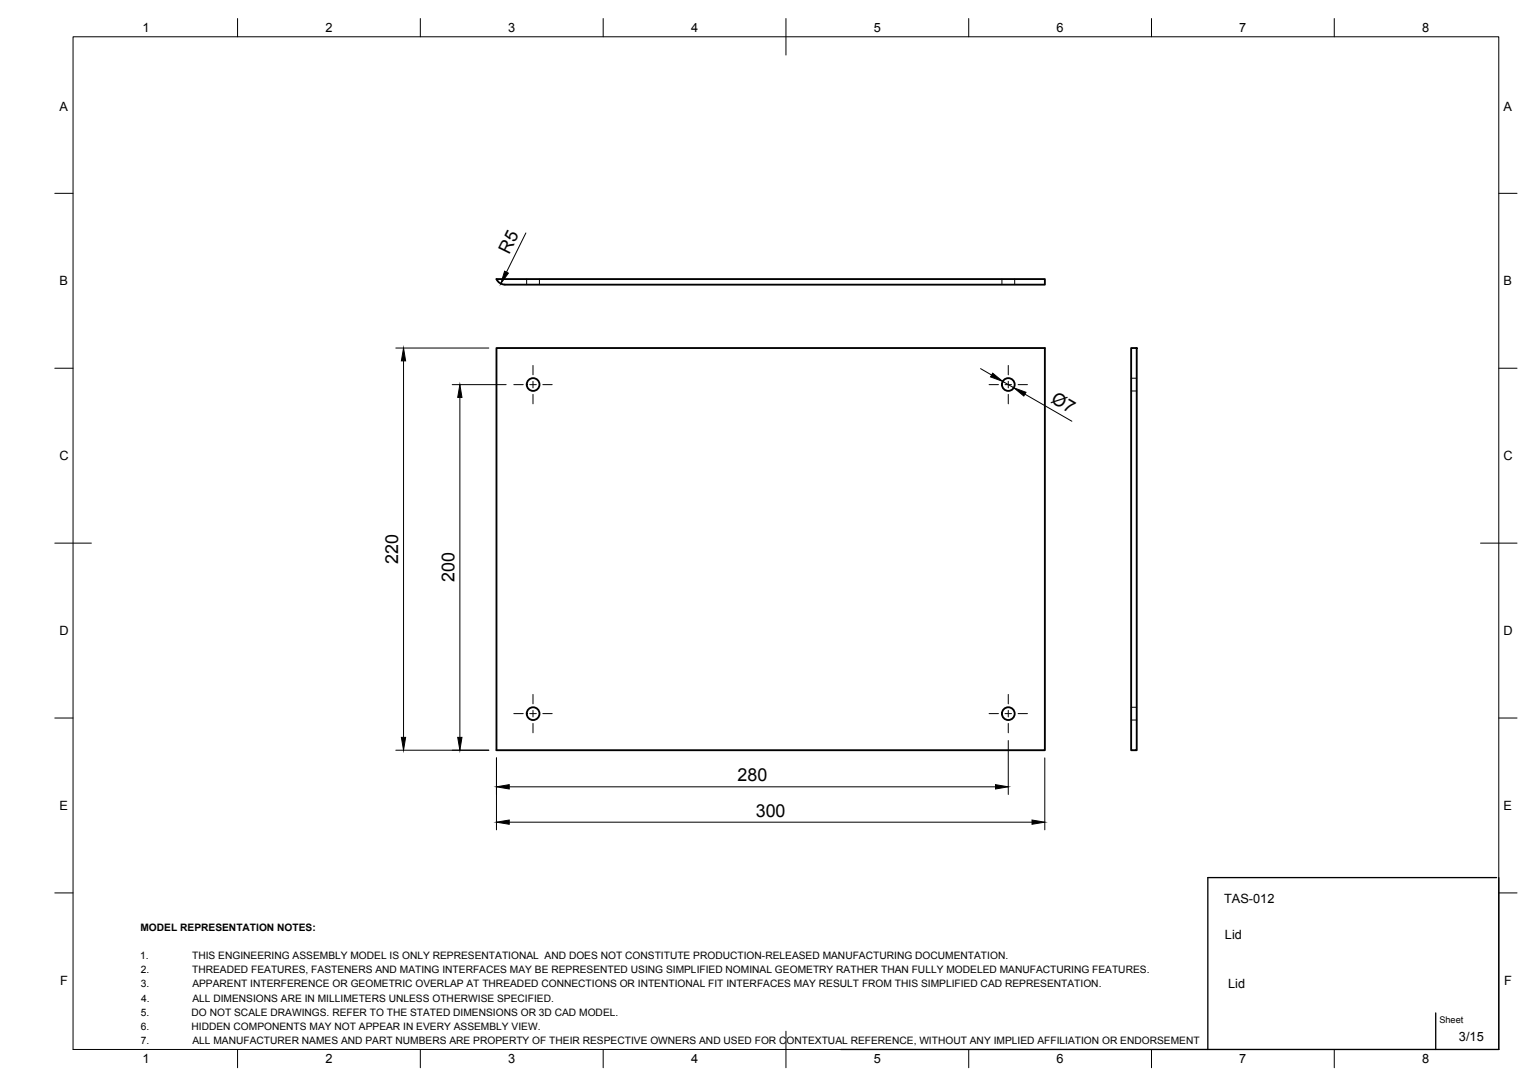
ISO-10303-21;
HEADER;
/* Generated by software containing ST-Developer
 * from STEP Tools, Inc. (www.steptools.com) 
 */

FILE_DESCRIPTION(
/* description */ (
'Independent welded steel electronics enclosure with removable sealed 
lid, internal mounting tray and two threaded cable entries. 300 x 220 
mm body. No ingress or electrical safety rating assigned.'),
/* implementation_level */ '2;1');

FILE_NAME(
/* name */ 'Lid.step',
/* time_stamp */ '2026-11-14T09:13:27-08:00',
/* author */ (''),
/* organization */ (''),
/* preprocessor_version */ 'ST-DEVELOPER v20.2',
/* originating_system */ 'Autodesk Translation Framework v15.17.0.0',
/* authorisation */ '');

FILE_SCHEMA (('AUTOMOTIVE_DESIGN { 1 0 10303 214 3 1 1 }'));
ENDSEC;

DATA;
#10=MECHANICAL_DESIGN_GEOMETRIC_PRESENTATION_REPRESENTATION('',(#973),#94412);
#943=SHAPE_REPRESENTATION_RELATIONSHIP('SRR','None',#94495,#958);
#958=ADVANCED_BREP_SHAPE_REPRESENTATION('',(#988),#94404);
#973=STYLED_ITEM('',(#94579),#988);
#988=MANIFOLD_SOLID_BREP('Body1',#8258);
#1017=FACE_BOUND('',#1741,.T.);
#1018=FACE_BOUND('',#1742,.T.);
#1019=FACE_BOUND('',#1743,.T.);
#1020=FACE_BOUND('',#1744,.T.);
#1021=FACE_BOUND('',#1753,.T.);
#1022=FACE_BOUND('',#1754,.T.);
#1023=FACE_BOUND('',#1755,.T.);
#1024=FACE_BOUND('',#1756,.T.);
#1110=PLANE('',#8714);
#1111=PLANE('',#8719);
#1112=PLANE('',#8728);
#1113=PLANE('',#8729);
#1114=PLANE('',#8730);
#1362=FACE_OUTER_BOUND('',#1739,.T.);
#1363=FACE_OUTER_BOUND('',#1740,.T.);
#1364=FACE_OUTER_BOUND('',#1745,.T.);
#1365=FACE_OUTER_BOUND('',#1746,.T.);
#1366=FACE_OUTER_BOUND('',#1747,.T.);
#1367=FACE_OUTER_BOUND('',#1748,.T.);
#1368=FACE_OUTER_BOUND('',#1749,.T.);
#1369=FACE_OUTER_BOUND('',#1750,.T.);
#1370=FACE_OUTER_BOUND('',#1751,.T.);
#1371=FACE_OUTER_BOUND('',#1752,.T.);
#1739=EDGE_LOOP('',(#6644,#6645,#6646,#6647));
#1740=EDGE_LOOP('',(#6648,#6649,#6650,#6651));
#1741=EDGE_LOOP('',(#6652));
#1742=EDGE_LOOP('',(#6653));
#1743=EDGE_LOOP('',(#6654));
#1744=EDGE_LOOP('',(#6655));
#1745=EDGE_LOOP('',(#6656,#6657,#6658,#6659));
#1746=EDGE_LOOP('',(#6660,#6661,#6662,#6663));
#1747=EDGE_LOOP('',(#6664,#6665,#6666,#6667));
#1748=EDGE_LOOP('',(#6668,#6669,#6670,#6671));
#1749=EDGE_LOOP('',(#6672,#6673,#6674,#6675));
#1750=EDGE_LOOP('',(#6676,#6677,#6678,#6679));
#1751=EDGE_LOOP('',(#6680,#6681,#6682,#6683));
#1752=EDGE_LOOP('',(#6684,#6685,#6686,#6687));
#1753=EDGE_LOOP('',(#6688));
#1754=EDGE_LOOP('',(#6689));
#1755=EDGE_LOOP('',(#6690));
#1756=EDGE_LOOP('',(#6691));
#2161=LINE('',#59703,#2559);
#2162=LINE('',#59706,#2560);
#2163=LINE('',#59709,#2561);
#2164=LINE('',#59711,#2562);
#2165=LINE('',#59712,#2563);
#2166=LINE('',#59723,#2564);
#2167=LINE('',#59724,#2565);
#2168=LINE('',#59727,#2566);
#2169=LINE('',#59731,#2567);
#2170=LINE('',#59735,#2568);
#2171=LINE('',#59739,#2569);
#2172=LINE('',#59743,#2570);
#2173=LINE('',#59744,#2571);
#2174=LINE('',#59746,#2572);
#2559=VECTOR('',#9733,5.);
#2560=VECTOR('',#9736,10.);
#2561=VECTOR('',#9739,10.);
#2562=VECTOR('',#9740,10.);
#2563=VECTOR('',#9741,10.);
#2564=VECTOR('',#9752,10.);
#2565=VECTOR('',#9753,10.);
#2566=VECTOR('',#9756,3.5);
#2567=VECTOR('',#9761,3.5);
#2568=VECTOR('',#9766,3.5);
#2569=VECTOR('',#9771,3.5);
#2570=VECTOR('',#9776,10.);
#2571=VECTOR('',#9777,10.);
#2572=VECTOR('',#9780,10.);
#2784=CIRCLE('',#8712,5.00000000000001);
#2785=CIRCLE('',#8713,5.00000000000001);
#2786=CIRCLE('',#8715,3.5);
#2787=CIRCLE('',#8716,3.5);
#2788=CIRCLE('',#8717,3.5);
#2789=CIRCLE('',#8718,3.5);
#2790=CIRCLE('',#8721,3.5);
#2791=CIRCLE('',#8723,3.5);
#2792=CIRCLE('',#8725,3.5);
#2793=CIRCLE('',#8727,3.5);
#3436=VERTEX_POINT('',#59699);
#3437=VERTEX_POINT('',#59700);
#3438=VERTEX_POINT('',#59702);
#3439=VERTEX_POINT('',#59704);
#3440=VERTEX_POINT('',#59708);
#3441=VERTEX_POINT('',#59710);
#3442=VERTEX_POINT('',#59713);
#3443=VERTEX_POINT('',#59715);
#3444=VERTEX_POINT('',#59717);
#3445=VERTEX_POINT('',#59719);
#3446=VERTEX_POINT('',#59722);
#3447=VERTEX_POINT('',#59726);
#3448=VERTEX_POINT('',#59730);
#3449=VERTEX_POINT('',#59734);
#3450=VERTEX_POINT('',#59738);
#3451=VERTEX_POINT('',#59742);
#4587=EDGE_CURVE('',#3436,#3437,#2784,.T.);
#4588=EDGE_CURVE('',#3437,#3438,#2161,.T.);
#4589=EDGE_CURVE('',#3438,#3439,#2785,.T.);
#4590=EDGE_CURVE('',#3439,#3436,#2162,.T.);
#4591=EDGE_CURVE('',#3437,#3440,#2163,.T.);
#4592=EDGE_CURVE('',#3440,#3441,#2164,.T.);
#4593=EDGE_CURVE('',#3441,#3438,#2165,.T.);
#4594=EDGE_CURVE('',#3442,#3442,#2786,.T.);
#4595=EDGE_CURVE('',#3443,#3443,#2787,.T.);
#4596=EDGE_CURVE('',#3444,#3444,#2788,.T.);
#4597=EDGE_CURVE('',#3445,#3445,#2789,.T.);
#4598=EDGE_CURVE('',#3436,#3446,#2166,.T.);
#4599=EDGE_CURVE('',#3446,#3440,#2167,.T.);
#4600=EDGE_CURVE('',#3445,#3447,#2168,.T.);
#4601=EDGE_CURVE('',#3447,#3447,#2790,.T.);
#4602=EDGE_CURVE('',#3444,#3448,#2169,.T.);
#4603=EDGE_CURVE('',#3448,#3448,#2791,.T.);
#4604=EDGE_CURVE('',#3443,#3449,#2170,.T.);
#4605=EDGE_CURVE('',#3449,#3449,#2792,.T.);
#4606=EDGE_CURVE('',#3442,#3450,#2171,.T.);
#4607=EDGE_CURVE('',#3450,#3450,#2793,.T.);
#4608=EDGE_CURVE('',#3451,#3441,#2172,.T.);
#4609=EDGE_CURVE('',#3451,#3439,#2173,.T.);
#4610=EDGE_CURVE('',#3446,#3451,#2174,.T.);
#6644=ORIENTED_EDGE('',*,*,#4587,.T.);
#6645=ORIENTED_EDGE('',*,*,#4588,.T.);
#6646=ORIENTED_EDGE('',*,*,#4589,.T.);
#6647=ORIENTED_EDGE('',*,*,#4590,.T.);
#6648=ORIENTED_EDGE('',*,*,#4588,.F.);
#6649=ORIENTED_EDGE('',*,*,#4591,.T.);
#6650=ORIENTED_EDGE('',*,*,#4592,.T.);
#6651=ORIENTED_EDGE('',*,*,#4593,.T.);
#6652=ORIENTED_EDGE('',*,*,#4594,.T.);
#6653=ORIENTED_EDGE('',*,*,#4595,.T.);
#6654=ORIENTED_EDGE('',*,*,#4596,.T.);
#6655=ORIENTED_EDGE('',*,*,#4597,.T.);
#6656=ORIENTED_EDGE('',*,*,#4587,.F.);
#6657=ORIENTED_EDGE('',*,*,#4598,.T.);
#6658=ORIENTED_EDGE('',*,*,#4599,.T.);
#6659=ORIENTED_EDGE('',*,*,#4591,.F.);
#6660=ORIENTED_EDGE('',*,*,#4597,.F.);
#6661=ORIENTED_EDGE('',*,*,#4600,.T.);
#6662=ORIENTED_EDGE('',*,*,#4601,.F.);
#6663=ORIENTED_EDGE('',*,*,#4600,.F.);
#6664=ORIENTED_EDGE('',*,*,#4596,.F.);
#6665=ORIENTED_EDGE('',*,*,#4602,.T.);
#6666=ORIENTED_EDGE('',*,*,#4603,.F.);
#6667=ORIENTED_EDGE('',*,*,#4602,.F.);
#6668=ORIENTED_EDGE('',*,*,#4595,.F.);
#6669=ORIENTED_EDGE('',*,*,#4604,.T.);
#6670=ORIENTED_EDGE('',*,*,#4605,.F.);
#6671=ORIENTED_EDGE('',*,*,#4604,.F.);
#6672=ORIENTED_EDGE('',*,*,#4594,.F.);
#6673=ORIENTED_EDGE('',*,*,#4606,.T.);
#6674=ORIENTED_EDGE('',*,*,#4607,.F.);
#6675=ORIENTED_EDGE('',*,*,#4606,.F.);
#6676=ORIENTED_EDGE('',*,*,#4589,.F.);
#6677=ORIENTED_EDGE('',*,*,#4593,.F.);
#6678=ORIENTED_EDGE('',*,*,#4608,.F.);
#6679=ORIENTED_EDGE('',*,*,#4609,.T.);
#6680=ORIENTED_EDGE('',*,*,#4610,.T.);
#6681=ORIENTED_EDGE('',*,*,#4608,.T.);
#6682=ORIENTED_EDGE('',*,*,#4592,.F.);
#6683=ORIENTED_EDGE('',*,*,#4599,.F.);
#6684=ORIENTED_EDGE('',*,*,#4610,.F.);
#6685=ORIENTED_EDGE('',*,*,#4598,.F.);
#6686=ORIENTED_EDGE('',*,*,#4590,.F.);
#6687=ORIENTED_EDGE('',*,*,#4609,.F.);
#6688=ORIENTED_EDGE('',*,*,#4601,.T.);
#6689=ORIENTED_EDGE('',*,*,#4603,.T.);
#6690=ORIENTED_EDGE('',*,*,#4605,.T.);
#6691=ORIENTED_EDGE('',*,*,#4607,.T.);
#7801=CYLINDRICAL_SURFACE('',#8711,5.00000000000001);
#7802=CYLINDRICAL_SURFACE('',#8720,3.5);
#7803=CYLINDRICAL_SURFACE('',#8722,3.5);
#7804=CYLINDRICAL_SURFACE('',#8724,3.5);
#7805=CYLINDRICAL_SURFACE('',#8726,3.5);
#8099=ADVANCED_FACE('',(#1362),#7801,.T.);
#8100=ADVANCED_FACE('',(#1363,#1017,#1018,#1019,#1020),#1110,.T.);
#8101=ADVANCED_FACE('',(#1364),#1111,.T.);
#8102=ADVANCED_FACE('',(#1365),#7802,.F.);
#8103=ADVANCED_FACE('',(#1366),#7803,.F.);
#8104=ADVANCED_FACE('',(#1367),#7804,.F.);
#8105=ADVANCED_FACE('',(#1368),#7805,.F.);
#8106=ADVANCED_FACE('',(#1369),#1112,.T.);
#8107=ADVANCED_FACE('',(#1370),#1113,.T.);
#8108=ADVANCED_FACE('',(#1371,#1021,#1022,#1023,#1024),#1114,.F.);
#8258=CLOSED_SHELL('',(#8099,#8100,#8101,#8102,#8103,#8104,#8105,#8106,
#8107,#8108));
#8710=AXIS2_PLACEMENT_3D('',#59697,#9727,#9728);
#8711=AXIS2_PLACEMENT_3D('',#59698,#9729,#9730);
#8712=AXIS2_PLACEMENT_3D('',#59701,#9731,#9732);
#8713=AXIS2_PLACEMENT_3D('',#59705,#9734,#9735);
#8714=AXIS2_PLACEMENT_3D('',#59707,#9737,#9738);
#8715=AXIS2_PLACEMENT_3D('',#59714,#9742,#9743);
#8716=AXIS2_PLACEMENT_3D('',#59716,#9744,#9745);
#8717=AXIS2_PLACEMENT_3D('',#59718,#9746,#9747);
#8718=AXIS2_PLACEMENT_3D('',#59720,#9748,#9749);
#8719=AXIS2_PLACEMENT_3D('',#59721,#9750,#9751);
#8720=AXIS2_PLACEMENT_3D('',#59725,#9754,#9755);
#8721=AXIS2_PLACEMENT_3D('',#59728,#9757,#9758);
#8722=AXIS2_PLACEMENT_3D('',#59729,#9759,#9760);
#8723=AXIS2_PLACEMENT_3D('',#59732,#9762,#9763);
#8724=AXIS2_PLACEMENT_3D('',#59733,#9764,#9765);
#8725=AXIS2_PLACEMENT_3D('',#59736,#9767,#9768);
#8726=AXIS2_PLACEMENT_3D('',#59737,#9769,#9770);
#8727=AXIS2_PLACEMENT_3D('',#59740,#9772,#9773);
#8728=AXIS2_PLACEMENT_3D('',#59741,#9774,#9775);
#8729=AXIS2_PLACEMENT_3D('',#59745,#9778,#9779);
#8730=AXIS2_PLACEMENT_3D('',#59747,#9781,#9782);
#9727=DIRECTION('axis',(0.,0.,1.));
#9728=DIRECTION('refdir',(1.,0.,0.));
#9729=DIRECTION('center_axis',(0.,-1.,0.));
#9730=DIRECTION('ref_axis',(0.916515138991168,0.,0.399999999999999));
#9731=DIRECTION('center_axis',(0.,-1.,0.));
#9732=DIRECTION('ref_axis',(0.916515138991168,0.,0.399999999999999));
#9733=DIRECTION('',(0.,-1.,0.));
#9734=DIRECTION('center_axis',(0.,1.,0.));
#9735=DIRECTION('ref_axis',(0.916515138991168,0.,0.399999999999999));
#9736=DIRECTION('',(0.,1.,0.));
#9737=DIRECTION('center_axis',(0.,0.,1.));
#9738=DIRECTION('ref_axis',(1.,0.,0.));
#9739=DIRECTION('',(-1.,0.,0.));
#9740=DIRECTION('',(0.,-1.,0.));
#9741=DIRECTION('',(1.,0.,0.));
#9742=DIRECTION('center_axis',(0.,0.,-1.));
#9743=DIRECTION('ref_axis',(1.,0.,0.));
#9744=DIRECTION('center_axis',(0.,0.,-1.));
#9745=DIRECTION('ref_axis',(1.,0.,0.));
#9746=DIRECTION('center_axis',(0.,0.,-1.));
#9747=DIRECTION('ref_axis',(1.,0.,0.));
#9748=DIRECTION('center_axis',(0.,0.,-1.));
#9749=DIRECTION('ref_axis',(1.,0.,0.));
#9750=DIRECTION('center_axis',(0.,1.,0.));
#9751=DIRECTION('ref_axis',(-1.,0.,0.));
#9752=DIRECTION('',(-1.,0.,0.));
#9753=DIRECTION('',(0.,0.,1.));
#9754=DIRECTION('center_axis',(0.,0.,-1.));
#9755=DIRECTION('ref_axis',(1.,0.,0.));
#9756=DIRECTION('',(0.,0.,-1.));
#9757=DIRECTION('center_axis',(0.,0.,1.));
#9758=DIRECTION('ref_axis',(1.,0.,0.));
#9759=DIRECTION('center_axis',(0.,0.,-1.));
#9760=DIRECTION('ref_axis',(1.,0.,0.));
#9761=DIRECTION('',(0.,0.,-1.));
#9762=DIRECTION('center_axis',(0.,0.,1.));
#9763=DIRECTION('ref_axis',(1.,0.,0.));
#9764=DIRECTION('center_axis',(0.,0.,-1.));
#9765=DIRECTION('ref_axis',(1.,0.,0.));
#9766=DIRECTION('',(0.,0.,-1.));
#9767=DIRECTION('center_axis',(0.,0.,1.));
#9768=DIRECTION('ref_axis',(1.,0.,0.));
#9769=DIRECTION('center_axis',(0.,0.,-1.));
#9770=DIRECTION('ref_axis',(1.,0.,0.));
#9771=DIRECTION('',(0.,0.,-1.));
#9772=DIRECTION('center_axis',(0.,0.,1.));
#9773=DIRECTION('ref_axis',(1.,0.,0.));
#9774=DIRECTION('center_axis',(0.,-1.,0.));
#9775=DIRECTION('ref_axis',(1.,0.,0.));
#9776=DIRECTION('',(0.,0.,1.));
#9777=DIRECTION('',(1.,0.,0.));
#9778=DIRECTION('center_axis',(-1.,0.,0.));
#9779=DIRECTION('ref_axis',(0.,-1.,0.));
#9780=DIRECTION('',(0.,-1.,0.));
#9781=DIRECTION('center_axis',(0.,0.,1.));
#9782=DIRECTION('ref_axis',(1.,0.,0.));
#59697=CARTESIAN_POINT('',(0.,0.,0.));
#59698=CARTESIAN_POINT('Origin',(145.417424305044,-110.,-2.));
#59699=CARTESIAN_POINT('',(150.,110.,0.));
#59700=CARTESIAN_POINT('',(145.417424305044,110.,3.));
#59701=CARTESIAN_POINT('Origin',(145.417424305044,110.,-2.));
#59702=CARTESIAN_POINT('',(145.417424305044,-110.,3.));
#59703=CARTESIAN_POINT('',(145.417424305044,-110.,3.));
#59704=CARTESIAN_POINT('',(150.,-110.,0.));
#59705=CARTESIAN_POINT('Origin',(145.417424305044,-110.,-2.));
#59706=CARTESIAN_POINT('',(150.,-110.,0.));
#59707=CARTESIAN_POINT('Origin',(0.,0.,3.));
#59708=CARTESIAN_POINT('',(-150.,110.,3.));
#59709=CARTESIAN_POINT('',(150.,110.,3.));
#59710=CARTESIAN_POINT('',(-150.,-110.,3.));
#59711=CARTESIAN_POINT('',(-150.,110.,3.));
#59712=CARTESIAN_POINT('',(-150.,-110.,3.));
#59713=CARTESIAN_POINT('',(126.5,90.,3.));
#59714=CARTESIAN_POINT('Origin',(130.,90.,3.));
#59715=CARTESIAN_POINT('',(-133.5,90.,3.));
#59716=CARTESIAN_POINT('Origin',(-130.,90.,3.));
#59717=CARTESIAN_POINT('',(-133.5,-90.,3.));
#59718=CARTESIAN_POINT('Origin',(-130.,-90.,3.));
#59719=CARTESIAN_POINT('',(126.5,-90.,3.));
#59720=CARTESIAN_POINT('Origin',(130.,-90.,3.));
#59721=CARTESIAN_POINT('Origin',(150.,110.,0.));
#59722=CARTESIAN_POINT('',(-150.,110.,0.));
#59723=CARTESIAN_POINT('',(150.,110.,0.));
#59724=CARTESIAN_POINT('',(-150.,110.,0.));
#59725=CARTESIAN_POINT('Origin',(130.,-90.,1.5));
#59726=CARTESIAN_POINT('',(126.5,-90.,0.));
#59727=CARTESIAN_POINT('',(126.5,-90.,1.5));
#59728=CARTESIAN_POINT('Origin',(130.,-90.,0.));
#59729=CARTESIAN_POINT('Origin',(-130.,-90.,1.5));
#59730=CARTESIAN_POINT('',(-133.5,-90.,0.));
#59731=CARTESIAN_POINT('',(-133.5,-90.,1.5));
#59732=CARTESIAN_POINT('Origin',(-130.,-90.,0.));
#59733=CARTESIAN_POINT('Origin',(-130.,90.,1.5));
#59734=CARTESIAN_POINT('',(-133.5,90.,0.));
#59735=CARTESIAN_POINT('',(-133.5,90.,1.5));
#59736=CARTESIAN_POINT('Origin',(-130.,90.,0.));
#59737=CARTESIAN_POINT('Origin',(130.,90.,1.5));
#59738=CARTESIAN_POINT('',(126.5,90.,0.));
#59739=CARTESIAN_POINT('',(126.5,90.,1.5));
#59740=CARTESIAN_POINT('Origin',(130.,90.,0.));
#59741=CARTESIAN_POINT('Origin',(-150.,-110.,0.));
#59742=CARTESIAN_POINT('',(-150.,-110.,0.));
#59743=CARTESIAN_POINT('',(-150.,-110.,0.));
#59744=CARTESIAN_POINT('',(-150.,-110.,0.));
#59745=CARTESIAN_POINT('Origin',(-150.,110.,0.));
#59746=CARTESIAN_POINT('',(-150.,110.,0.));
#59747=CARTESIAN_POINT('Origin',(0.,0.,0.));
#94386=UNCERTAINTY_MEASURE_WITH_UNIT(LENGTH_MEASURE(0.01),#94413,
'DISTANCE_ACCURACY_VALUE',
'Maximum model space distance between geometric entities at asserted c
onnectivities');
#94394=UNCERTAINTY_MEASURE_WITH_UNIT(LENGTH_MEASURE(0.01),#94413,
'DISTANCE_ACCURACY_VALUE',
'Maximum model space distance between geometric entities at asserted c
onnectivities');
#94404=(
GEOMETRIC_REPRESENTATION_CONTEXT(3)
GLOBAL_UNCERTAINTY_ASSIGNED_CONTEXT((#94386))
GLOBAL_UNIT_ASSIGNED_CONTEXT((#94413,#94415,#94416))
REPRESENTATION_CONTEXT('','3D')
);
#94412=(
GEOMETRIC_REPRESENTATION_CONTEXT(3)
GLOBAL_UNCERTAINTY_ASSIGNED_CONTEXT((#94394))
GLOBAL_UNIT_ASSIGNED_CONTEXT((#94413,#94415,#94416))
REPRESENTATION_CONTEXT('','3D')
);
#94413=(
LENGTH_UNIT()
NAMED_UNIT(*)
SI_UNIT(.MILLI.,.METRE.)
);
#94415=(
NAMED_UNIT(*)
PLANE_ANGLE_UNIT()
SI_UNIT($,.RADIAN.)
);
#94416=(
NAMED_UNIT(*)
SI_UNIT($,.STERADIAN.)
SOLID_ANGLE_UNIT()
);
#94426=SHAPE_DEFINITION_REPRESENTATION(#94460,#94495);
#94460=PRODUCT_DEFINITION_SHAPE('',$,#94513);
#94495=SHAPE_REPRESENTATION('',(#8710),#94404);
#94503=PRODUCT_DEFINITION_CONTEXT('part definition',#94556,'design');
#94513=PRODUCT_DEFINITION('Lid','Lid',#94530,#94503);
#94530=PRODUCT_DEFINITION_FORMATION('',$,#94567);
#94556=APPLICATION_CONTEXT(
'Core Data for Automotive Mechanical Design Process');
#94557=PRODUCT_CONTEXT('part definition',#94556,'mechanical');
#94567=PRODUCT('Lid','Lid',$,(#94557));
#94579=PRESENTATION_STYLE_ASSIGNMENT((#94586));
#94586=SURFACE_STYLE_USAGE(.BOTH.,#94593);
#94593=SURFACE_SIDE_STYLE('',(#94600));
#94600=SURFACE_STYLE_FILL_AREA(#94607);
#94607=FILL_AREA_STYLE('Opaque(169,212,242)',(#94614));
#94614=FILL_AREA_STYLE_COLOUR('Opaque(169,212,242)',#94621);
#94621=COLOUR_RGB('Opaque(169,212,242)',0.662745098039216,0.831372549019608,
0.949019607843137);
ENDSEC;
END-ISO-10303-21;
